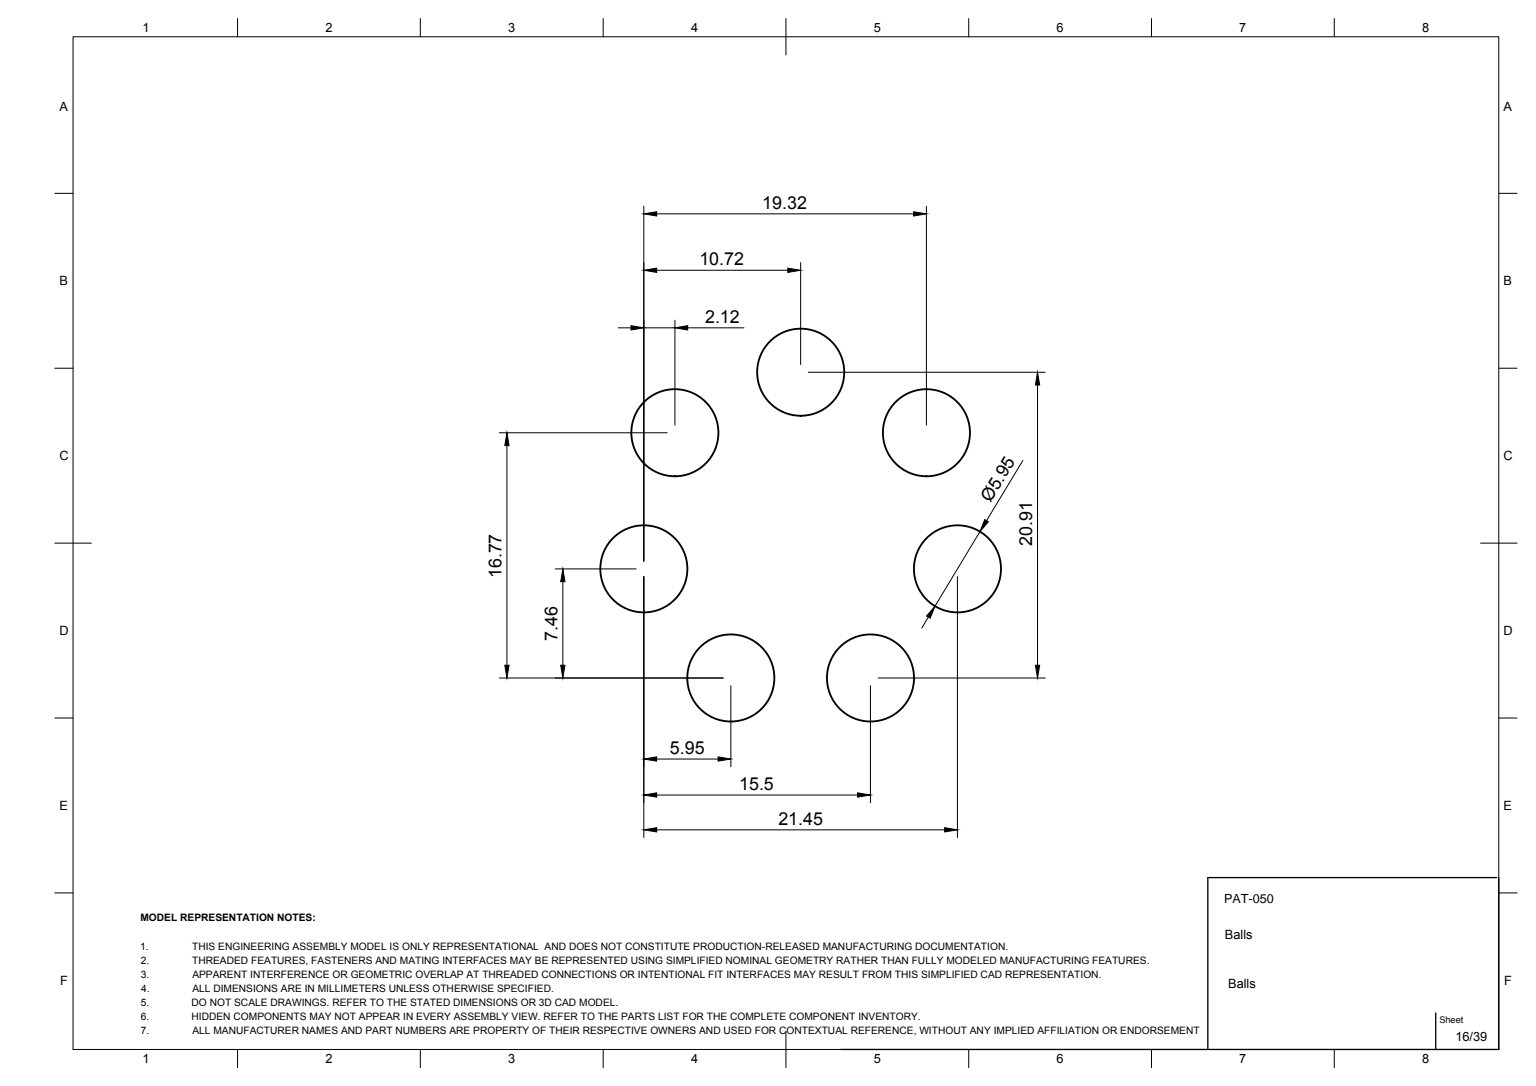
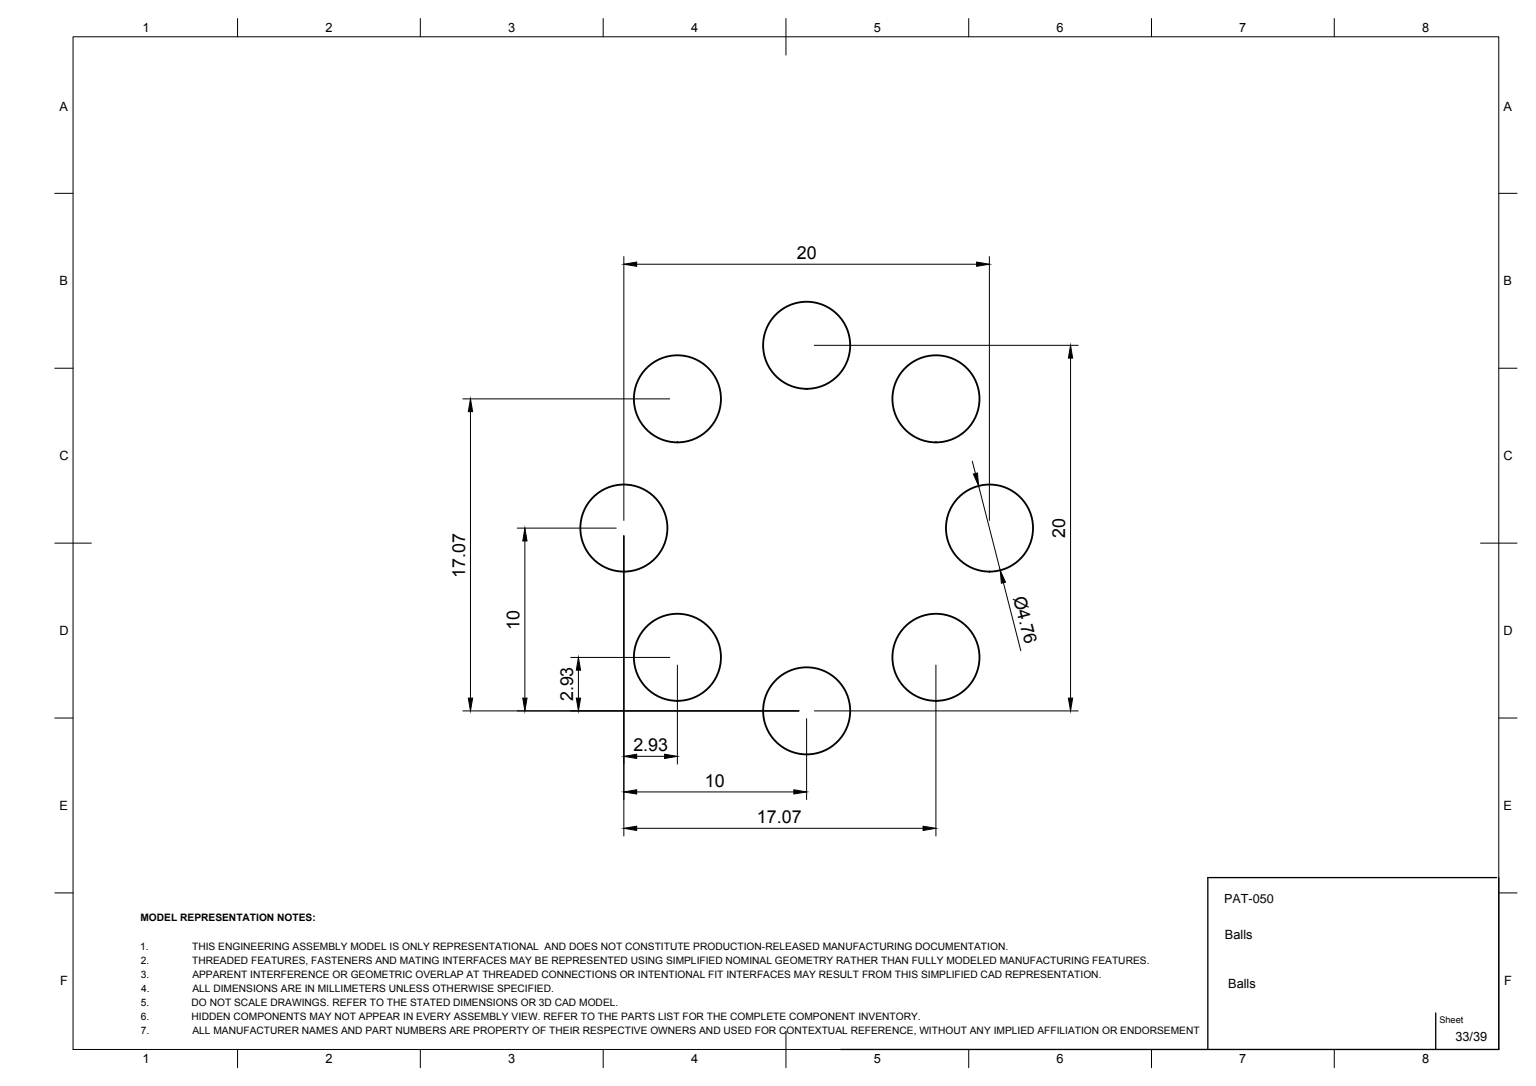
ISO-10303-21;
HEADER;
/* Generated by software containing ST-Developer
 * from STEP Tools, Inc. (www.steptools.com) 
 */

FILE_DESCRIPTION(
/* description */ ('Hand wheel with handle and shaft collar'),
/* implementation_level */ '2;1');

FILE_NAME(
/* name */ 'Balls.step',
/* time_stamp */ '2026-10-28T03:23:19-07:00',
/* author */ (''),
/* organization */ (''),
/* preprocessor_version */ 'ST-DEVELOPER v20.2',
/* originating_system */ 'Autodesk Translation Framework v15.17.0.0',
/* authorisation */ '');

FILE_SCHEMA (('AUTOMOTIVE_DESIGN { 1 0 10303 214 3 1 1 }'));
ENDSEC;

DATA;
#10=MECHANICAL_DESIGN_GEOMETRIC_PRESENTATION_REPRESENTATION('',(#406,#407,#408,#409,#410,#411,#412),#10510);
#267=SPHERICAL_SURFACE('',#5904,0.29765);
#268=SPHERICAL_SURFACE('',#5906,0.29765);
#269=SPHERICAL_SURFACE('',#5908,0.29765);
#270=SPHERICAL_SURFACE('',#5910,0.29765);
#271=SPHERICAL_SURFACE('',#5912,0.29765);
#272=SPHERICAL_SURFACE('',#5914,0.29765);
#273=SPHERICAL_SURFACE('',#5916,0.29765);
#342=SHAPE_REPRESENTATION_RELATIONSHIP('SRR','None',#10659,#374);
#374=ADVANCED_BREP_SHAPE_REPRESENTATION('',(#452,#453,#454,#455,#456,#457,
#458),#10486);
#406=STYLED_ITEM('',(#10908),#452);
#407=STYLED_ITEM('',(#10908),#453);
#408=STYLED_ITEM('',(#10908),#454);
#409=STYLED_ITEM('',(#10908),#455);
#410=STYLED_ITEM('',(#10908),#456);
#411=STYLED_ITEM('',(#10908),#457);
#412=STYLED_ITEM('',(#10908),#458);
#452=MANIFOLD_SOLID_BREP('Body1',#5306);
#453=MANIFOLD_SOLID_BREP('Body2',#5307);
#454=MANIFOLD_SOLID_BREP('Body3',#5308);
#455=MANIFOLD_SOLID_BREP('Body4',#5309);
#456=MANIFOLD_SOLID_BREP('Body5',#5310);
#457=MANIFOLD_SOLID_BREP('Body6',#5311);
#458=MANIFOLD_SOLID_BREP('Body7',#5312);
#864=FACE_OUTER_BOUND('',#1240,.T.);
#865=FACE_OUTER_BOUND('',#1241,.T.);
#866=FACE_OUTER_BOUND('',#1242,.T.);
#867=FACE_OUTER_BOUND('',#1243,.T.);
#868=FACE_OUTER_BOUND('',#1244,.T.);
#869=FACE_OUTER_BOUND('',#1245,.T.);
#870=FACE_OUTER_BOUND('',#1246,.T.);
#1240=EDGE_LOOP('',(#3987,#3988));
#1241=EDGE_LOOP('',(#3989,#3990));
#1242=EDGE_LOOP('',(#3991,#3992));
#1243=EDGE_LOOP('',(#3993,#3994));
#1244=EDGE_LOOP('',(#3995,#3996));
#1245=EDGE_LOOP('',(#3997,#3998));
#1246=EDGE_LOOP('',(#3999,#4000));
#2224=CIRCLE('',#5905,0.29765);
#2225=CIRCLE('',#5907,0.29765);
#2226=CIRCLE('',#5909,0.29765);
#2227=CIRCLE('',#5911,0.29765);
#2228=CIRCLE('',#5913,0.29765);
#2229=CIRCLE('',#5915,0.29765);
#2230=CIRCLE('',#5917,0.29765);
#2585=VERTEX_POINT('',#8646);
#2586=VERTEX_POINT('',#8647);
#2587=VERTEX_POINT('',#8650);
#2588=VERTEX_POINT('',#8651);
#2589=VERTEX_POINT('',#8654);
#2590=VERTEX_POINT('',#8655);
#2591=VERTEX_POINT('',#8658);
#2592=VERTEX_POINT('',#8659);
#2593=VERTEX_POINT('',#8662);
#2594=VERTEX_POINT('',#8663);
#2595=VERTEX_POINT('',#8666);
#2596=VERTEX_POINT('',#8667);
#2597=VERTEX_POINT('',#8670);
#2598=VERTEX_POINT('',#8671);
#3111=EDGE_CURVE('',#2585,#2586,#2224,.T.);
#3112=EDGE_CURVE('',#2587,#2588,#2225,.T.);
#3113=EDGE_CURVE('',#2589,#2590,#2226,.T.);
#3114=EDGE_CURVE('',#2591,#2592,#2227,.T.);
#3115=EDGE_CURVE('',#2593,#2594,#2228,.T.);
#3116=EDGE_CURVE('',#2595,#2596,#2229,.T.);
#3117=EDGE_CURVE('',#2597,#2598,#2230,.T.);
#3987=ORIENTED_EDGE('',*,*,#3111,.T.);
#3988=ORIENTED_EDGE('',*,*,#3111,.F.);
#3989=ORIENTED_EDGE('',*,*,#3112,.T.);
#3990=ORIENTED_EDGE('',*,*,#3112,.F.);
#3991=ORIENTED_EDGE('',*,*,#3113,.T.);
#3992=ORIENTED_EDGE('',*,*,#3113,.F.);
#3993=ORIENTED_EDGE('',*,*,#3114,.T.);
#3994=ORIENTED_EDGE('',*,*,#3114,.F.);
#3995=ORIENTED_EDGE('',*,*,#3115,.T.);
#3996=ORIENTED_EDGE('',*,*,#3115,.F.);
#3997=ORIENTED_EDGE('',*,*,#3116,.T.);
#3998=ORIENTED_EDGE('',*,*,#3116,.F.);
#3999=ORIENTED_EDGE('',*,*,#3117,.T.);
#4000=ORIENTED_EDGE('',*,*,#3117,.F.);
#5076=ADVANCED_FACE('',(#864),#267,.T.);
#5077=ADVANCED_FACE('',(#865),#268,.T.);
#5078=ADVANCED_FACE('',(#866),#269,.T.);
#5079=ADVANCED_FACE('',(#867),#270,.T.);
#5080=ADVANCED_FACE('',(#868),#271,.T.);
#5081=ADVANCED_FACE('',(#869),#272,.T.);
#5082=ADVANCED_FACE('',(#870),#273,.T.);
#5306=CLOSED_SHELL('',(#5076));
#5307=CLOSED_SHELL('',(#5077));
#5308=CLOSED_SHELL('',(#5078));
#5309=CLOSED_SHELL('',(#5079));
#5310=CLOSED_SHELL('',(#5080));
#5311=CLOSED_SHELL('',(#5081));
#5312=CLOSED_SHELL('',(#5082));
#5903=AXIS2_PLACEMENT_3D('',#8644,#6955,#6956);
#5904=AXIS2_PLACEMENT_3D('',#8645,#6957,#6958);
#5905=AXIS2_PLACEMENT_3D('',#8648,#6959,#6960);
#5906=AXIS2_PLACEMENT_3D('',#8649,#6961,#6962);
#5907=AXIS2_PLACEMENT_3D('',#8652,#6963,#6964);
#5908=AXIS2_PLACEMENT_3D('',#8653,#6965,#6966);
#5909=AXIS2_PLACEMENT_3D('',#8656,#6967,#6968);
#5910=AXIS2_PLACEMENT_3D('',#8657,#6969,#6970);
#5911=AXIS2_PLACEMENT_3D('',#8660,#6971,#6972);
#5912=AXIS2_PLACEMENT_3D('',#8661,#6973,#6974);
#5913=AXIS2_PLACEMENT_3D('',#8664,#6975,#6976);
#5914=AXIS2_PLACEMENT_3D('',#8665,#6977,#6978);
#5915=AXIS2_PLACEMENT_3D('',#8668,#6979,#6980);
#5916=AXIS2_PLACEMENT_3D('',#8669,#6981,#6982);
#5917=AXIS2_PLACEMENT_3D('',#8672,#6983,#6984);
#6955=DIRECTION('axis',(0.,0.,1.));
#6956=DIRECTION('refdir',(1.,0.,0.));
#6957=DIRECTION('center_axis',(0.,0.,1.));
#6958=DIRECTION('ref_axis',(1.,0.,0.));
#6959=DIRECTION('center_axis',(1.22464679914735E-16,-1.,0.));
#6960=DIRECTION('ref_axis',(-1.,-1.22464679914735E-16,0.));
#6961=DIRECTION('center_axis',(0.78183148246803,0.,0.623489801858733));
#6962=DIRECTION('ref_axis',(0.623489801858734,0.,-0.78183148246803));
#6963=DIRECTION('center_axis',(7.63554790147315E-17,-1.,-9.57467422477103E-17));
#6964=DIRECTION('ref_axis',(-0.623489801858734,-1.22464679914735E-16,0.78183148246803));
#6965=DIRECTION('center_axis',(0.974927912181824,0.,-0.222520933956314));
#6966=DIRECTION('ref_axis',(-0.222520933956314,0.,-0.974927912181824));
#6967=DIRECTION('center_axis',(-2.7250954951288E-17,-1.,-1.19394234705288E-16));
#6968=DIRECTION('ref_axis',(0.222520933956314,-1.22464679914735E-16,0.974927912181824));
#6969=DIRECTION('center_axis',(0.433883739117558,0.,-0.900968867902419));
#6970=DIRECTION('ref_axis',(-0.900968867902419,0.,-0.433883739117558));
#6971=DIRECTION('center_axis',(-1.10336864020811E-16,-1.,-5.31354332312403E-17));
#6972=DIRECTION('ref_axis',(0.900968867902419,-1.22464679914735E-16,0.433883739117558));
#6973=DIRECTION('center_axis',(-0.433883739117558,0.,-0.900968867902419));
#6974=DIRECTION('ref_axis',(-0.900968867902419,0.,0.433883739117558));
#6975=DIRECTION('center_axis',(-1.10336864020811E-16,-1.,5.31354332312403E-17));
#6976=DIRECTION('ref_axis',(0.900968867902419,-1.22464679914735E-16,-0.433883739117558));
#6977=DIRECTION('center_axis',(-0.974927912181824,0.,-0.222520933956314));
#6978=DIRECTION('ref_axis',(-0.222520933956315,0.,0.974927912181824));
#6979=DIRECTION('center_axis',(-2.7250954951288E-17,-1.,1.19394234705288E-16));
#6980=DIRECTION('ref_axis',(0.222520933956315,-1.22464679914735E-16,-0.974927912181824));
#6981=DIRECTION('center_axis',(-0.78183148246803,0.,0.623489801858734));
#6982=DIRECTION('ref_axis',(0.623489801858733,0.,0.78183148246803));
#6983=DIRECTION('center_axis',(7.63554790147315E-17,-1.,9.57467422477103E-17));
#6984=DIRECTION('ref_axis',(-0.623489801858733,-1.22464679914735E-16,-0.78183148246803));
#8644=CARTESIAN_POINT('',(0.,0.,0.));
#8645=CARTESIAN_POINT('Origin',(1.1,0.,0.));
#8646=CARTESIAN_POINT('',(1.1,-2.23201749654651E-33,0.29765));
#8647=CARTESIAN_POINT('',(1.1,-2.23201749654651E-33,-0.29765));
#8648=CARTESIAN_POINT('Origin',(1.1,0.,0.));
#8649=CARTESIAN_POINT('Origin',(0.685838782044607,0.,-0.860014630714833));
#8650=CARTESIAN_POINT('',(0.918550922801216,-5.31350540756609E-33,-0.674432891191581));
#8651=CARTESIAN_POINT('',(0.453126641287998,8.49470414473068E-34,-1.04559637023808));
#8652=CARTESIAN_POINT('Origin',(0.685838782044607,0.,-0.860014630714833));
#8653=CARTESIAN_POINT('Origin',(-0.244773027351946,0.,-1.07242070340001));
#8654=CARTESIAN_POINT('',(0.0454142657089739,-2.23201749654651E-33,-1.1386540593921));
#8655=CARTESIAN_POINT('',(-0.534960320412865,-2.23201749654651E-33,-1.00618734740791));
#8656=CARTESIAN_POINT('Origin',(-0.244773027351946,0.,-1.07242070340001));
#8657=CARTESIAN_POINT('Origin',(-0.991065754692661,0.,-0.477272113029314));
#8658=CARTESIAN_POINT('',(-0.86192025974432,8.49470414473067E-34,-0.745445496560469));
#8659=CARTESIAN_POINT('',(-1.120211249641,-5.31350540756609E-33,-0.209098729498159));
#8660=CARTESIAN_POINT('Origin',(-0.991065754692661,0.,-0.477272113029314));
#8661=CARTESIAN_POINT('Origin',(-0.991065754692661,0.,0.477272113029314));
#8662=CARTESIAN_POINT('',(-1.120211249641,-2.23201749654651E-33,0.209098729498159));
#8663=CARTESIAN_POINT('',(-0.86192025974432,-2.23201749654651E-33,0.745445496560469));
#8664=CARTESIAN_POINT('Origin',(-0.991065754692661,0.,0.477272113029314));
#8665=CARTESIAN_POINT('Origin',(-0.244773027351946,0.,1.07242070340001));
#8666=CARTESIAN_POINT('',(-0.534960320412866,-2.23201749654651E-33,1.00618734740791));
#8667=CARTESIAN_POINT('',(0.0454142657089737,-2.23201749654651E-33,1.1386540593921));
#8668=CARTESIAN_POINT('Origin',(-0.244773027351946,0.,1.07242070340001));
#8669=CARTESIAN_POINT('Origin',(0.685838782044607,0.,0.860014630714833));
#8670=CARTESIAN_POINT('',(0.453126641287998,-2.23201749654651E-33,1.04559637023808));
#8671=CARTESIAN_POINT('',(0.918550922801216,-2.23201749654651E-33,0.674432891191581));
#8672=CARTESIAN_POINT('Origin',(0.685838782044607,0.,0.860014630714833));
#10447=UNCERTAINTY_MEASURE_WITH_UNIT(LENGTH_MEASURE(0.001),#10511,
'DISTANCE_ACCURACY_VALUE',
'Maximum model space distance between geometric entities at asserted c
onnectivities');
#10471=UNCERTAINTY_MEASURE_WITH_UNIT(LENGTH_MEASURE(0.001),#10511,
'DISTANCE_ACCURACY_VALUE',
'Maximum model space distance between geometric entities at asserted c
onnectivities');
#10486=(
GEOMETRIC_REPRESENTATION_CONTEXT(3)
GLOBAL_UNCERTAINTY_ASSIGNED_CONTEXT((#10447))
GLOBAL_UNIT_ASSIGNED_CONTEXT((#10511,#10513,#10514))
REPRESENTATION_CONTEXT('','3D')
);
#10510=(
GEOMETRIC_REPRESENTATION_CONTEXT(3)
GLOBAL_UNCERTAINTY_ASSIGNED_CONTEXT((#10471))
GLOBAL_UNIT_ASSIGNED_CONTEXT((#10511,#10513,#10514))
REPRESENTATION_CONTEXT('','3D')
);
#10511=(
LENGTH_UNIT()
NAMED_UNIT(*)
SI_UNIT(.CENTI.,.METRE.)
);
#10513=(
NAMED_UNIT(*)
PLANE_ANGLE_UNIT()
SI_UNIT($,.RADIAN.)
);
#10514=(
NAMED_UNIT(*)
SI_UNIT($,.STERADIAN.)
SOLID_ANGLE_UNIT()
);
#10529=SHAPE_DEFINITION_REPRESENTATION(#10567,#10659);
#10567=PRODUCT_DEFINITION_SHAPE('',$,#10698);
#10659=SHAPE_REPRESENTATION('',(#5903),#10486);
#10683=PRODUCT_DEFINITION_CONTEXT('part definition',#10799,'design');
#10698=PRODUCT_DEFINITION('Balls','Balls',#10736,#10683);
#10736=PRODUCT_DEFINITION_FORMATION('',$,#10815);
#10799=APPLICATION_CONTEXT(
'Core Data for Automotive Mechanical Design Process');
#10800=PRODUCT_CONTEXT('part definition',#10799,'mechanical');
#10815=PRODUCT('Balls','Balls','Balls',(#10800));
#10902=COLOUR_RGB('Grey',0.48,0.52,0.57);
#10903=FILL_AREA_STYLE_COLOUR('',#10902);
#10904=FILL_AREA_STYLE('',(#10903));
#10905=SURFACE_STYLE_FILL_AREA(#10904);
#10906=SURFACE_SIDE_STYLE('',(#10905));
#10907=SURFACE_STYLE_USAGE(.BOTH.,#10906);
#10908=PRESENTATION_STYLE_ASSIGNMENT((#10907));
ENDSEC;
END-ISO-10303-21;
